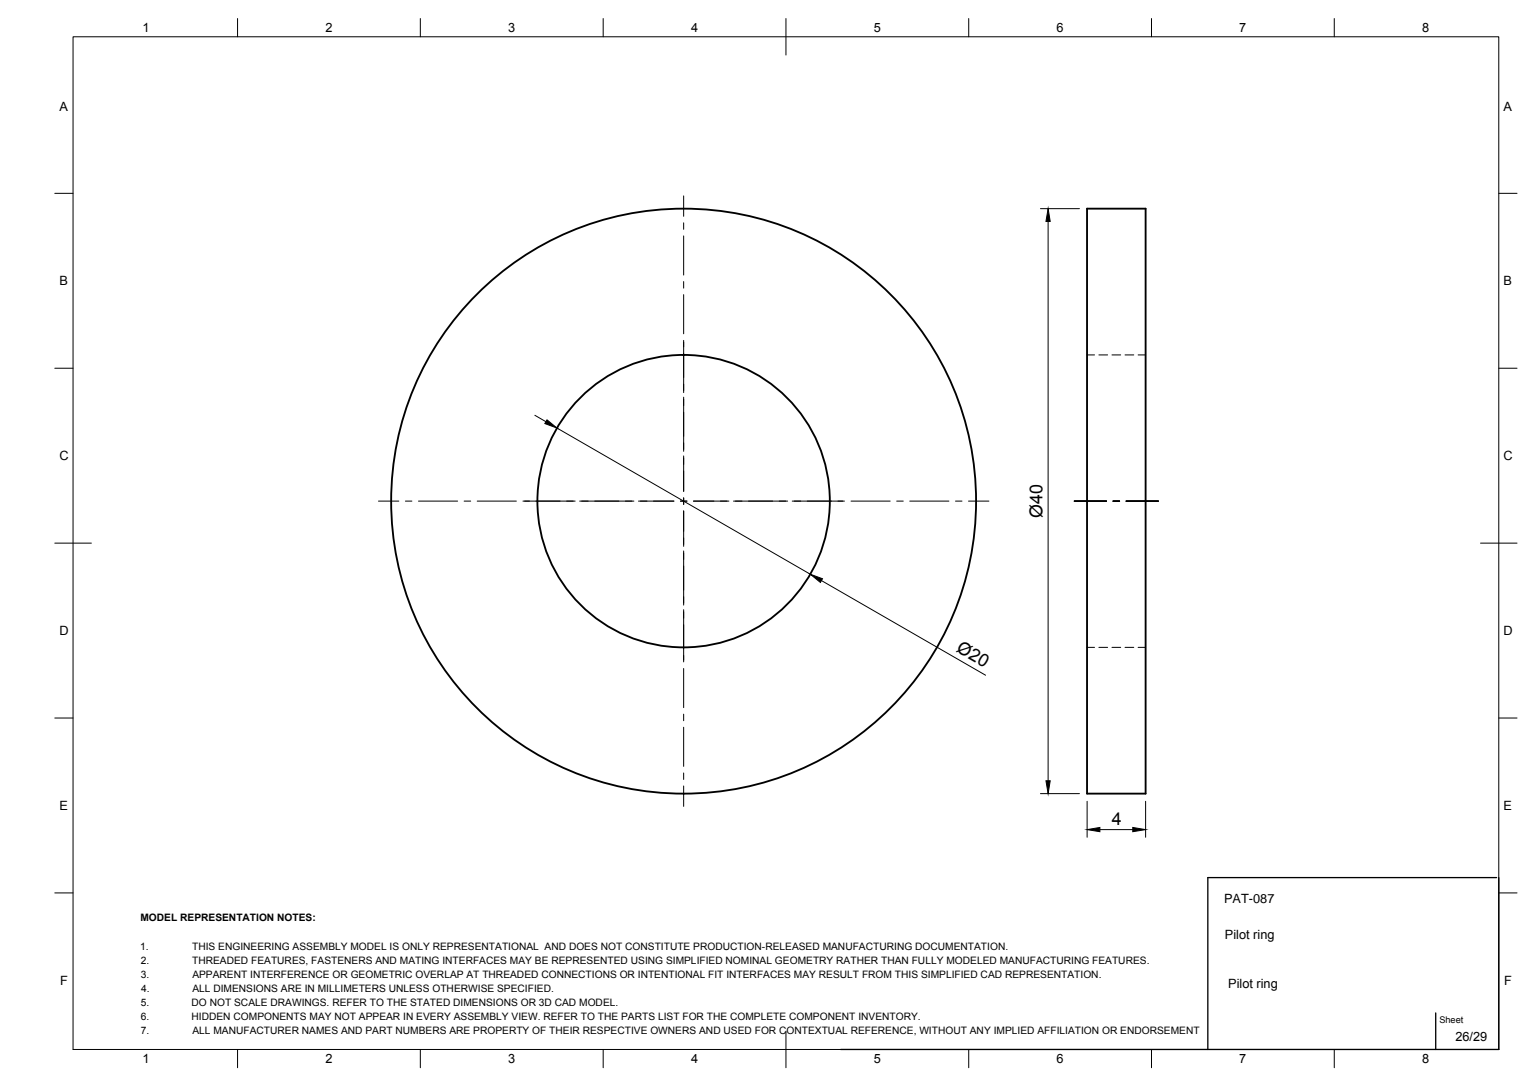
ISO-10303-21;
HEADER;
/* Generated by software containing ST-Developer
 * from STEP Tools, Inc. (www.steptools.com) 
 */

FILE_DESCRIPTION(
/* description */ ('Rigid flange shaft coupling assembly'),
/* implementation_level */ '2;1');

FILE_NAME(
/* name */ 'Pilot ring.step',
/* time_stamp */ '2026-10-27T10:47:16-07:00',
/* author */ (''),
/* organization */ (''),
/* preprocessor_version */ 'ST-DEVELOPER v20.2',
/* originating_system */ 'Autodesk Translation Framework v15.17.0.0',
/* authorisation */ '');

FILE_SCHEMA (('AUTOMOTIVE_DESIGN { 1 0 10303 214 3 1 1 }'));
ENDSEC;

DATA;
#10=MECHANICAL_DESIGN_GEOMETRIC_PRESENTATION_REPRESENTATION('',(#418),#9141);
#361=SHAPE_REPRESENTATION_RELATIONSHIP('SRR','None',#9297,#389);
#389=ADVANCED_BREP_SHAPE_REPRESENTATION('',(#446),#9132);
#418=STYLED_ITEM('',(#9493),#446);
#446=MANIFOLD_SOLID_BREP('Body1',#4773);
#553=FACE_BOUND('',#1302,.T.);
#554=FACE_BOUND('',#1304,.T.);
#683=PLANE('',#5443);
#684=PLANE('',#5444);
#927=FACE_OUTER_BOUND('',#1299,.T.);
#928=FACE_OUTER_BOUND('',#1300,.T.);
#929=FACE_OUTER_BOUND('',#1301,.T.);
#930=FACE_OUTER_BOUND('',#1303,.T.);
#1299=EDGE_LOOP('',(#4035,#4036,#4037,#4038));
#1300=EDGE_LOOP('',(#4039,#4040,#4041,#4042));
#1301=EDGE_LOOP('',(#4043));
#1302=EDGE_LOOP('',(#4044));
#1303=EDGE_LOOP('',(#4045));
#1304=EDGE_LOOP('',(#4046));
#1634=LINE('',#8477,#1979);
#1635=LINE('',#8483,#1980);
#1979=VECTOR('',#6563,1.);
#1980=VECTOR('',#6570,2.);
#2230=CIRCLE('',#5438,1.);
#2231=CIRCLE('',#5439,1.);
#2232=CIRCLE('',#5441,2.);
#2233=CIRCLE('',#5442,2.);
#2547=VERTEX_POINT('',#8474);
#2548=VERTEX_POINT('',#8476);
#2549=VERTEX_POINT('',#8480);
#2550=VERTEX_POINT('',#8482);
#3061=EDGE_CURVE('',#2547,#2547,#2230,.T.);
#3062=EDGE_CURVE('',#2547,#2548,#1634,.T.);
#3063=EDGE_CURVE('',#2548,#2548,#2231,.T.);
#3064=EDGE_CURVE('',#2549,#2549,#2232,.T.);
#3065=EDGE_CURVE('',#2549,#2550,#1635,.T.);
#3066=EDGE_CURVE('',#2550,#2550,#2233,.T.);
#4035=ORIENTED_EDGE('',*,*,#3061,.F.);
#4036=ORIENTED_EDGE('',*,*,#3062,.T.);
#4037=ORIENTED_EDGE('',*,*,#3063,.T.);
#4038=ORIENTED_EDGE('',*,*,#3062,.F.);
#4039=ORIENTED_EDGE('',*,*,#3064,.F.);
#4040=ORIENTED_EDGE('',*,*,#3065,.T.);
#4041=ORIENTED_EDGE('',*,*,#3066,.T.);
#4042=ORIENTED_EDGE('',*,*,#3065,.F.);
#4043=ORIENTED_EDGE('',*,*,#3064,.T.);
#4044=ORIENTED_EDGE('',*,*,#3061,.T.);
#4045=ORIENTED_EDGE('',*,*,#3066,.F.);
#4046=ORIENTED_EDGE('',*,*,#3063,.F.);
#4464=CYLINDRICAL_SURFACE('',#5437,1.);
#4465=CYLINDRICAL_SURFACE('',#5440,2.);
#4663=ADVANCED_FACE('',(#927),#4464,.F.);
#4664=ADVANCED_FACE('',(#928),#4465,.T.);
#4665=ADVANCED_FACE('',(#929,#553),#683,.T.);
#4666=ADVANCED_FACE('',(#930,#554),#684,.F.);
#4773=CLOSED_SHELL('',(#4663,#4664,#4665,#4666));
#5436=AXIS2_PLACEMENT_3D('',#8472,#6557,#6558);
#5437=AXIS2_PLACEMENT_3D('',#8473,#6559,#6560);
#5438=AXIS2_PLACEMENT_3D('',#8475,#6561,#6562);
#5439=AXIS2_PLACEMENT_3D('',#8478,#6564,#6565);
#5440=AXIS2_PLACEMENT_3D('',#8479,#6566,#6567);
#5441=AXIS2_PLACEMENT_3D('',#8481,#6568,#6569);
#5442=AXIS2_PLACEMENT_3D('',#8484,#6571,#6572);
#5443=AXIS2_PLACEMENT_3D('',#8485,#6573,#6574);
#5444=AXIS2_PLACEMENT_3D('',#8486,#6575,#6576);
#6557=DIRECTION('axis',(0.,0.,1.));
#6558=DIRECTION('refdir',(1.,0.,0.));
#6559=DIRECTION('center_axis',(0.,1.,0.));
#6560=DIRECTION('ref_axis',(1.,0.,0.));
#6561=DIRECTION('center_axis',(0.,-1.,0.));
#6562=DIRECTION('ref_axis',(1.,0.,0.));
#6563=DIRECTION('',(0.,-1.,0.));
#6564=DIRECTION('center_axis',(0.,-1.,0.));
#6565=DIRECTION('ref_axis',(1.,0.,0.));
#6566=DIRECTION('center_axis',(0.,1.,0.));
#6567=DIRECTION('ref_axis',(1.,0.,0.));
#6568=DIRECTION('center_axis',(0.,1.,0.));
#6569=DIRECTION('ref_axis',(1.,0.,0.));
#6570=DIRECTION('',(0.,-1.,0.));
#6571=DIRECTION('center_axis',(0.,1.,0.));
#6572=DIRECTION('ref_axis',(1.,0.,0.));
#6573=DIRECTION('center_axis',(0.,1.,0.));
#6574=DIRECTION('ref_axis',(1.,0.,0.));
#6575=DIRECTION('center_axis',(0.,1.,0.));
#6576=DIRECTION('ref_axis',(1.,0.,0.));
#8472=CARTESIAN_POINT('',(0.,0.,0.));
#8473=CARTESIAN_POINT('Origin',(0.,9.8,6.53));
#8474=CARTESIAN_POINT('',(-1.,10.2,6.53));
#8475=CARTESIAN_POINT('Origin',(0.,10.2,6.53));
#8476=CARTESIAN_POINT('',(-1.,9.8,6.53));
#8477=CARTESIAN_POINT('',(-1.,9.8,6.53));
#8478=CARTESIAN_POINT('Origin',(0.,9.8,6.53));
#8479=CARTESIAN_POINT('Origin',(0.,9.8,6.53));
#8480=CARTESIAN_POINT('',(-2.,10.2,6.53));
#8481=CARTESIAN_POINT('Origin',(0.,10.2,6.53));
#8482=CARTESIAN_POINT('',(-2.,9.8,6.53));
#8483=CARTESIAN_POINT('',(-2.,9.8,6.53));
#8484=CARTESIAN_POINT('Origin',(0.,9.8,6.53));
#8485=CARTESIAN_POINT('Origin',(0.,10.2,6.53));
#8486=CARTESIAN_POINT('Origin',(0.,9.8,6.53));
#9099=UNCERTAINTY_MEASURE_WITH_UNIT(LENGTH_MEASURE(0.001),#9142,
'DISTANCE_ACCURACY_VALUE',
'Maximum model space distance between geometric entities at asserted c
onnectivities');
#9108=UNCERTAINTY_MEASURE_WITH_UNIT(LENGTH_MEASURE(0.001),#9142,
'DISTANCE_ACCURACY_VALUE',
'Maximum model space distance between geometric entities at asserted c
onnectivities');
#9132=(
GEOMETRIC_REPRESENTATION_CONTEXT(3)
GLOBAL_UNCERTAINTY_ASSIGNED_CONTEXT((#9099))
GLOBAL_UNIT_ASSIGNED_CONTEXT((#9142,#9144,#9145))
REPRESENTATION_CONTEXT('','3D')
);
#9141=(
GEOMETRIC_REPRESENTATION_CONTEXT(3)
GLOBAL_UNCERTAINTY_ASSIGNED_CONTEXT((#9108))
GLOBAL_UNIT_ASSIGNED_CONTEXT((#9142,#9144,#9145))
REPRESENTATION_CONTEXT('','3D')
);
#9142=(
LENGTH_UNIT()
NAMED_UNIT(*)
SI_UNIT(.CENTI.,.METRE.)
);
#9144=(
NAMED_UNIT(*)
PLANE_ANGLE_UNIT()
SI_UNIT($,.RADIAN.)
);
#9145=(
NAMED_UNIT(*)
SI_UNIT($,.STERADIAN.)
SOLID_ANGLE_UNIT()
);
#9169=SHAPE_DEFINITION_REPRESENTATION(#9203,#9297);
#9203=PRODUCT_DEFINITION_SHAPE('',$,#9330);
#9297=SHAPE_REPRESENTATION('',(#5436),#9132);
#9306=PRODUCT_DEFINITION_CONTEXT('part definition',#9404,'design');
#9330=PRODUCT_DEFINITION('Pilot ring','Pilot ring',#9362,#9306);
#9362=PRODUCT_DEFINITION_FORMATION('',$,#9429);
#9404=APPLICATION_CONTEXT(
'Core Data for Automotive Mechanical Design Process');
#9405=PRODUCT_CONTEXT('part definition',#9404,'mechanical');
#9429=PRODUCT('Pilot ring','Pilot ring','Pilot ring',(#9405));
#9487=COLOUR_RGB('Sky Blue',0.24,0.69,0.87);
#9488=FILL_AREA_STYLE_COLOUR('',#9487);
#9489=FILL_AREA_STYLE('',(#9488));
#9490=SURFACE_STYLE_FILL_AREA(#9489);
#9491=SURFACE_SIDE_STYLE('',(#9490));
#9492=SURFACE_STYLE_USAGE(.BOTH.,#9491);
#9493=PRESENTATION_STYLE_ASSIGNMENT((#9492));
ENDSEC;
END-ISO-10303-21;
